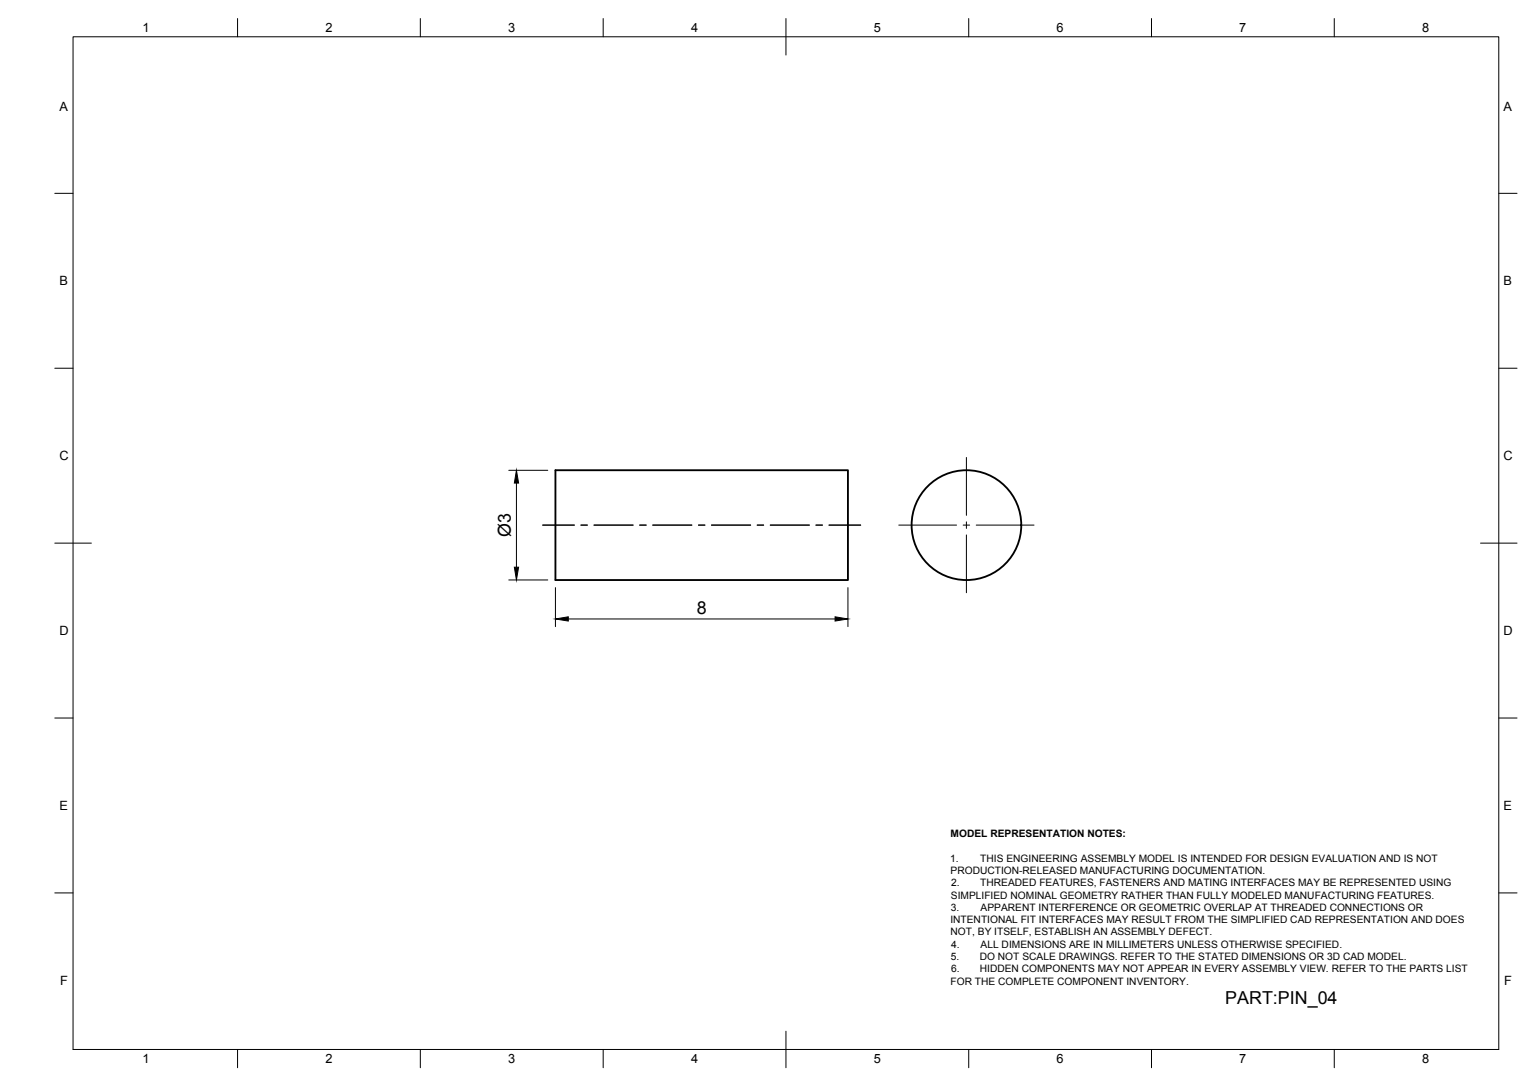
ISO-10303-21;
HEADER;
/* Generated by software containing ST-Developer
 * from STEP Tools, Inc. (www.steptools.com) 
 */

FILE_DESCRIPTION(
/* description */ (''),
/* implementation_level */ '2;1');

FILE_NAME(
/* name */ 'Pin_04.step',
/* time_stamp */ '2026-10-05T13:12:53-07:00',
/* author */ (''),
/* organization */ (''),
/* preprocessor_version */ 'ST-DEVELOPER v20.2',
/* originating_system */ 'Autodesk Translation Framework v15.15.0.0',
/* authorisation */ '');

FILE_SCHEMA (('AUTOMOTIVE_DESIGN { 1 0 10303 214 3 1 1 }'));
ENDSEC;

DATA;
#10=MECHANICAL_DESIGN_GEOMETRIC_PRESENTATION_REPRESENTATION('',(#63),#5912);
#47=SHAPE_REPRESENTATION_RELATIONSHIP('SRR','None',#5948,#55);
#55=ADVANCED_BREP_SHAPE_REPRESENTATION('',(#71),#5908);
#63=STYLED_ITEM('',(#5994),#71);
#71=MANIFOLD_SOLID_BREP('Body1',#3474);
#164=CYLINDRICAL_SURFACE('',#3855,1.50000013517123);
#338=FACE_OUTER_BOUND('',#541,.T.);
#339=FACE_OUTER_BOUND('',#542,.T.);
#340=FACE_OUTER_BOUND('',#543,.T.);
#541=EDGE_LOOP('',(#3136,#3137,#3138,#3139));
#542=EDGE_LOOP('',(#3140));
#543=EDGE_LOOP('',(#3141));
#647=CIRCLE('',#3856,1.50000013517123);
#648=CIRCLE('',#3857,1.50000013517123);
#1016=LINE('',#5854,#1381);
#1381=VECTOR('',#4827,1.50000013517123);
#1697=VERTEX_POINT('',#5851);
#1698=VERTEX_POINT('',#5853);
#2178=EDGE_CURVE('',#1697,#1697,#647,.T.);
#2179=EDGE_CURVE('',#1697,#1698,#1016,.T.);
#2180=EDGE_CURVE('',#1698,#1698,#648,.T.);
#3136=ORIENTED_EDGE('',*,*,#2178,.F.);
#3137=ORIENTED_EDGE('',*,*,#2179,.T.);
#3138=ORIENTED_EDGE('',*,*,#2180,.F.);
#3139=ORIENTED_EDGE('',*,*,#2179,.F.);
#3140=ORIENTED_EDGE('',*,*,#2180,.T.);
#3141=ORIENTED_EDGE('',*,*,#2178,.T.);
#3280=PLANE('',#3858);
#3281=PLANE('',#3859);
#3458=ADVANCED_FACE('',(#338),#164,.T.);
#3459=ADVANCED_FACE('',(#339),#3280,.T.);
#3460=ADVANCED_FACE('',(#340),#3281,.F.);
#3474=CLOSED_SHELL('',(#3458,#3459,#3460));
#3854=AXIS2_PLACEMENT_3D('',#5849,#4821,#4822);
#3855=AXIS2_PLACEMENT_3D('',#5850,#4823,#4824);
#3856=AXIS2_PLACEMENT_3D('',#5852,#4825,#4826);
#3857=AXIS2_PLACEMENT_3D('',#5855,#4828,#4829);
#3858=AXIS2_PLACEMENT_3D('',#5856,#4830,#4831);
#3859=AXIS2_PLACEMENT_3D('',#5857,#4832,#4833);
#4821=DIRECTION('axis',(0.,0.,1.));
#4822=DIRECTION('refdir',(1.,0.,0.));
#4823=DIRECTION('center_axis',(0.,-1.,0.));
#4824=DIRECTION('ref_axis',(-1.,0.,0.));
#4825=DIRECTION('center_axis',(1.83667601732677E-48,-1.,2.73691106313441E-48));
#4826=DIRECTION('ref_axis',(-1.,-1.83667601732677E-48,0.));
#4827=DIRECTION('',(0.,1.,0.));
#4828=DIRECTION('center_axis',(-1.83667601732677E-48,1.,-2.73691106313441E-48));
#4829=DIRECTION('ref_axis',(-1.,-1.83667601732677E-48,0.));
#4830=DIRECTION('center_axis',(-1.83667601732677E-48,1.,-2.73691106313441E-48));
#4831=DIRECTION('ref_axis',(-1.,-1.83667601732677E-48,0.));
#4832=DIRECTION('center_axis',(-1.83667601732677E-48,1.,-2.73691106313441E-48));
#4833=DIRECTION('ref_axis',(-1.,-1.83667601732677E-48,0.));
#5849=CARTESIAN_POINT('',(0.,0.,0.));
#5850=CARTESIAN_POINT('Origin',(10.0000020566038,-4.00000000000001,2.50000086324266));
#5851=CARTESIAN_POINT('',(11.500002191775,-12.,2.50000086324266));
#5852=CARTESIAN_POINT('Origin',(10.0000020566038,-12.,2.50000086324266));
#5853=CARTESIAN_POINT('',(11.500002191775,-4.00000000000001,2.50000086324266));
#5854=CARTESIAN_POINT('',(11.500002191775,-4.00000000000001,2.50000086324266));
#5855=CARTESIAN_POINT('Origin',(10.0000020566038,-4.00000000000001,2.50000086324266));
#5856=CARTESIAN_POINT('Origin',(10.0000020566038,-4.00000000000001,2.50000086324266));
#5857=CARTESIAN_POINT('Origin',(10.0000020566038,-12.,2.50000086324266));
#5898=UNCERTAINTY_MEASURE_WITH_UNIT(LENGTH_MEASURE(0.01),#5913,
'DISTANCE_ACCURACY_VALUE',
'Maximum model space distance between geometric entities at asserted c
onnectivities');
#5902=UNCERTAINTY_MEASURE_WITH_UNIT(LENGTH_MEASURE(0.01),#5913,
'DISTANCE_ACCURACY_VALUE',
'Maximum model space distance between geometric entities at asserted c
onnectivities');
#5908=(
GEOMETRIC_REPRESENTATION_CONTEXT(3)
GLOBAL_UNCERTAINTY_ASSIGNED_CONTEXT((#5898))
GLOBAL_UNIT_ASSIGNED_CONTEXT((#5913,#5915,#5916))
REPRESENTATION_CONTEXT('','3D')
);
#5912=(
GEOMETRIC_REPRESENTATION_CONTEXT(3)
GLOBAL_UNCERTAINTY_ASSIGNED_CONTEXT((#5902))
GLOBAL_UNIT_ASSIGNED_CONTEXT((#5913,#5915,#5916))
REPRESENTATION_CONTEXT('','3D')
);
#5913=(
LENGTH_UNIT()
NAMED_UNIT(*)
SI_UNIT(.MILLI.,.METRE.)
);
#5915=(
NAMED_UNIT(*)
PLANE_ANGLE_UNIT()
SI_UNIT($,.RADIAN.)
);
#5916=(
NAMED_UNIT(*)
SI_UNIT($,.STERADIAN.)
SOLID_ANGLE_UNIT()
);
#5922=SHAPE_DEFINITION_REPRESENTATION(#5931,#5948);
#5931=PRODUCT_DEFINITION_SHAPE('',$,#5958);
#5948=SHAPE_REPRESENTATION('',(#3854),#5908);
#5952=PRODUCT_DEFINITION_CONTEXT('part definition',#5981,'design');
#5958=PRODUCT_DEFINITION('Pin_04','Pin_04',#5967,#5952);
#5967=PRODUCT_DEFINITION_FORMATION('',$,#5988);
#5981=APPLICATION_CONTEXT(
'Core Data for Automotive Mechanical Design Process');
#5982=PRODUCT_CONTEXT('part definition',#5981,'mechanical');
#5988=PRODUCT('Pin_04','Pin_04',$,(#5982));
#5994=PRESENTATION_STYLE_ASSIGNMENT((#5997));
#5997=SURFACE_STYLE_USAGE(.BOTH.,#6000);
#6000=SURFACE_SIDE_STYLE('',(#6003));
#6003=SURFACE_STYLE_FILL_AREA(#6006);
#6006=FILL_AREA_STYLE('Opaque(160,160,160)',(#6009));
#6009=FILL_AREA_STYLE_COLOUR('Opaque(160,160,160)',#6012);
#6012=COLOUR_RGB('Opaque(160,160,160)', 0.31764706, 0.68627451, 0.89019608);
ENDSEC;
END-ISO-10303-21;
